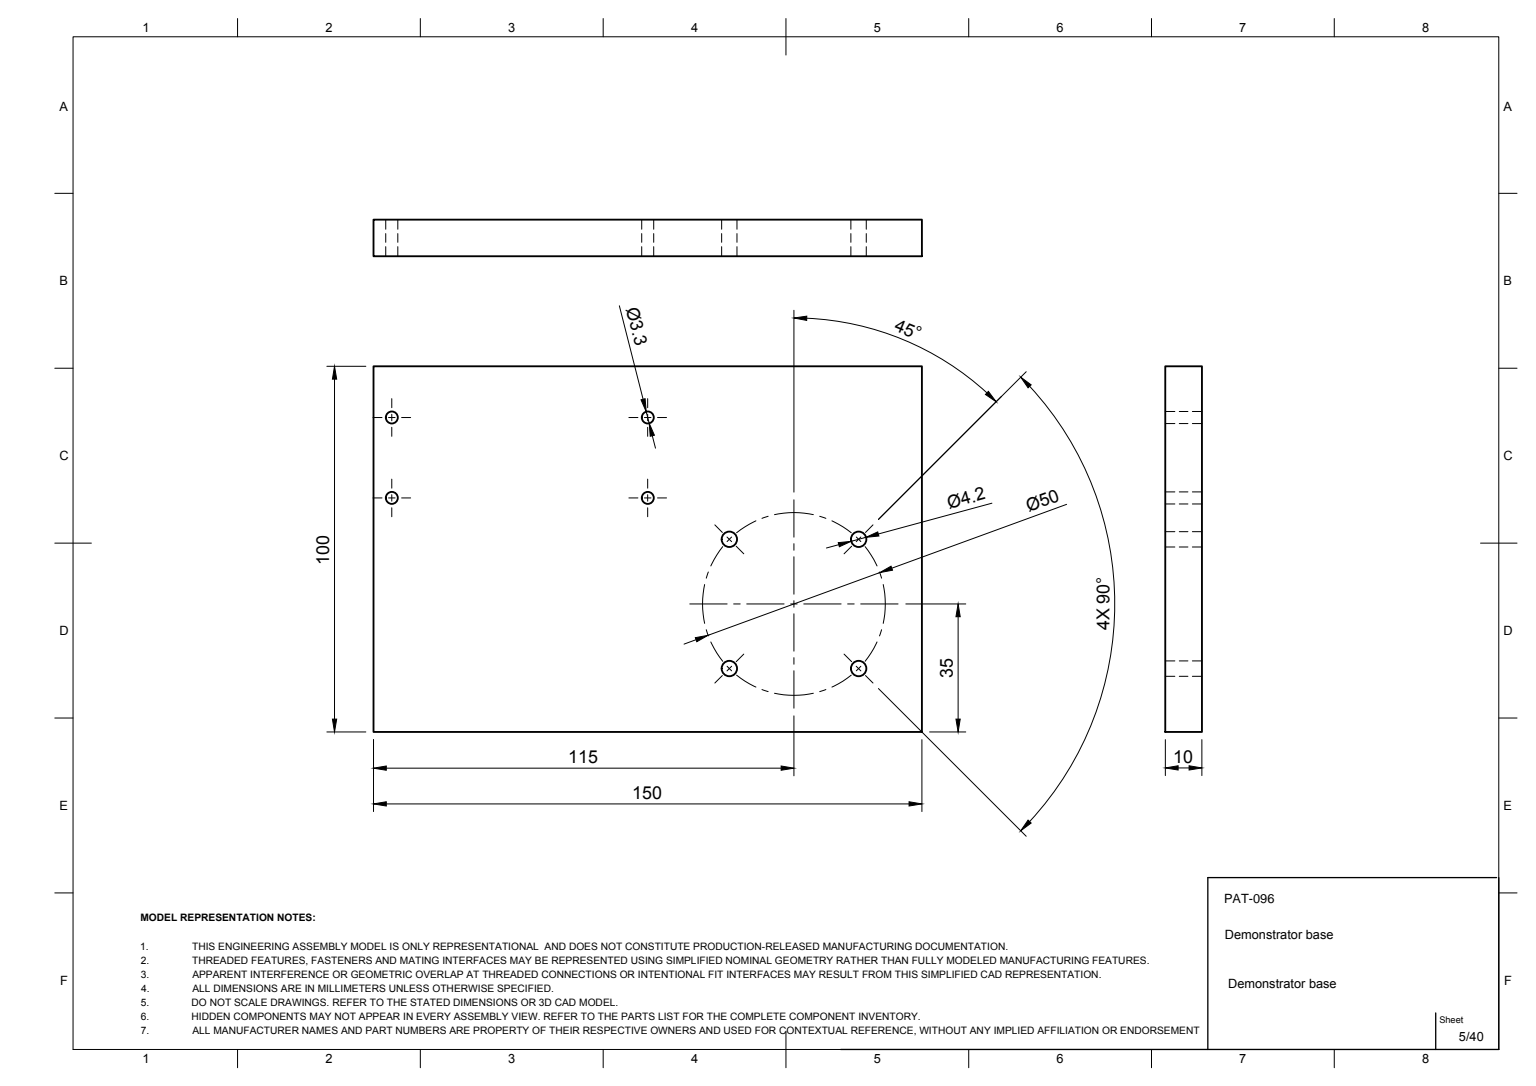
ISO-10303-21;
HEADER;
/* Generated by software containing ST-Developer
 * from STEP Tools, Inc. (www.steptools.com) 
 */

FILE_DESCRIPTION(
/* description */ ('PAT-096'),
/* implementation_level */ '2;1');

FILE_NAME(
/* name */ 'Demonstrator base.step',
/* time_stamp */ '2026-10-29T17:03:14-07:00',
/* author */ (''),
/* organization */ (''),
/* preprocessor_version */ 'ST-DEVELOPER v20.2',
/* originating_system */ 'Autodesk Translation Framework v15.17.0.0',
/* authorisation */ '');

FILE_SCHEMA (('AUTOMOTIVE_DESIGN { 1 0 10303 214 3 1 1 }'));
ENDSEC;

DATA;
#10=MECHANICAL_DESIGN_GEOMETRIC_PRESENTATION_REPRESENTATION('',(#398),#10650);
#336=SHAPE_REPRESENTATION_RELATIONSHIP('SRR','None',#10796,#367);
#367=ADVANCED_BREP_SHAPE_REPRESENTATION('',(#437),#10614);
#398=STYLED_ITEM('',(#11043),#437);
#437=MANIFOLD_SOLID_BREP('Body1',#5531);
#473=FACE_BOUND('',#1139,.T.);
#474=FACE_BOUND('',#1140,.T.);
#475=FACE_BOUND('',#1141,.T.);
#476=FACE_BOUND('',#1142,.T.);
#477=FACE_BOUND('',#1143,.T.);
#478=FACE_BOUND('',#1144,.T.);
#479=FACE_BOUND('',#1145,.T.);
#480=FACE_BOUND('',#1146,.T.);
#481=FACE_BOUND('',#1148,.T.);
#482=FACE_BOUND('',#1149,.T.);
#483=FACE_BOUND('',#1150,.T.);
#484=FACE_BOUND('',#1151,.T.);
#485=FACE_BOUND('',#1152,.T.);
#486=FACE_BOUND('',#1153,.T.);
#487=FACE_BOUND('',#1154,.T.);
#488=FACE_BOUND('',#1155,.T.);
#612=PLANE('',#5942);
#613=PLANE('',#5943);
#614=PLANE('',#5944);
#615=PLANE('',#5945);
#616=PLANE('',#5946);
#617=PLANE('',#5947);
#790=FACE_OUTER_BOUND('',#1126,.T.);
#791=FACE_OUTER_BOUND('',#1127,.T.);
#792=FACE_OUTER_BOUND('',#1128,.T.);
#793=FACE_OUTER_BOUND('',#1129,.T.);
#794=FACE_OUTER_BOUND('',#1130,.T.);
#795=FACE_OUTER_BOUND('',#1131,.T.);
#796=FACE_OUTER_BOUND('',#1132,.T.);
#797=FACE_OUTER_BOUND('',#1133,.T.);
#798=FACE_OUTER_BOUND('',#1134,.T.);
#799=FACE_OUTER_BOUND('',#1135,.T.);
#800=FACE_OUTER_BOUND('',#1136,.T.);
#801=FACE_OUTER_BOUND('',#1137,.T.);
#802=FACE_OUTER_BOUND('',#1138,.T.);
#803=FACE_OUTER_BOUND('',#1147,.T.);
#1126=EDGE_LOOP('',(#3715,#3716,#3717,#3718));
#1127=EDGE_LOOP('',(#3719,#3720,#3721,#3722));
#1128=EDGE_LOOP('',(#3723,#3724,#3725,#3726));
#1129=EDGE_LOOP('',(#3727,#3728,#3729,#3730));
#1130=EDGE_LOOP('',(#3731,#3732,#3733,#3734));
#1131=EDGE_LOOP('',(#3735,#3736,#3737,#3738));
#1132=EDGE_LOOP('',(#3739,#3740,#3741,#3742));
#1133=EDGE_LOOP('',(#3743,#3744,#3745,#3746));
#1134=EDGE_LOOP('',(#3747,#3748,#3749,#3750));
#1135=EDGE_LOOP('',(#3751,#3752,#3753,#3754));
#1136=EDGE_LOOP('',(#3755,#3756,#3757,#3758));
#1137=EDGE_LOOP('',(#3759,#3760,#3761,#3762));
#1138=EDGE_LOOP('',(#3763,#3764,#3765,#3766));
#1139=EDGE_LOOP('',(#3767));
#1140=EDGE_LOOP('',(#3768));
#1141=EDGE_LOOP('',(#3769));
#1142=EDGE_LOOP('',(#3770));
#1143=EDGE_LOOP('',(#3771));
#1144=EDGE_LOOP('',(#3772));
#1145=EDGE_LOOP('',(#3773));
#1146=EDGE_LOOP('',(#3774));
#1147=EDGE_LOOP('',(#3775,#3776,#3777,#3778));
#1148=EDGE_LOOP('',(#3779));
#1149=EDGE_LOOP('',(#3780));
#1150=EDGE_LOOP('',(#3781));
#1151=EDGE_LOOP('',(#3782));
#1152=EDGE_LOOP('',(#3783));
#1153=EDGE_LOOP('',(#3784));
#1154=EDGE_LOOP('',(#3785));
#1155=EDGE_LOOP('',(#3786));
#1601=LINE('',#8519,#1930);
#1602=LINE('',#8525,#1931);
#1603=LINE('',#8531,#1932);
#1604=LINE('',#8537,#1933);
#1605=LINE('',#8543,#1934);
#1606=LINE('',#8549,#1935);
#1607=LINE('',#8555,#1936);
#1608=LINE('',#8561,#1937);
#1609=LINE('',#8566,#1938);
#1610=LINE('',#8568,#1939);
#1611=LINE('',#8570,#1940);
#1612=LINE('',#8571,#1941);
#1613=LINE('',#8574,#1942);
#1614=LINE('',#8576,#1943);
#1615=LINE('',#8577,#1944);
#1616=LINE('',#8580,#1945);
#1617=LINE('',#8582,#1946);
#1618=LINE('',#8583,#1947);
#1619=LINE('',#8585,#1948);
#1620=LINE('',#8586,#1949);
#1930=VECTOR('',#6681,0.164999999999999);
#1931=VECTOR('',#6688,0.164999999999999);
#1932=VECTOR('',#6695,0.165);
#1933=VECTOR('',#6702,0.165);
#1934=VECTOR('',#6709,0.21);
#1935=VECTOR('',#6716,0.21);
#1936=VECTOR('',#6723,0.21);
#1937=VECTOR('',#6730,0.21);
#1938=VECTOR('',#6735,1.);
#1939=VECTOR('',#6736,1.);
#1940=VECTOR('',#6737,1.);
#1941=VECTOR('',#6738,1.);
#1942=VECTOR('',#6741,1.);
#1943=VECTOR('',#6742,1.);
#1944=VECTOR('',#6743,1.);
#1945=VECTOR('',#6746,1.);
#1946=VECTOR('',#6747,1.);
#1947=VECTOR('',#6748,1.);
#1948=VECTOR('',#6751,1.);
#1949=VECTOR('',#6752,1.);
#2259=CIRCLE('',#5919,0.164999999999999);
#2260=CIRCLE('',#5920,0.164999999999999);
#2261=CIRCLE('',#5922,0.164999999999999);
#2262=CIRCLE('',#5923,0.164999999999999);
#2263=CIRCLE('',#5925,0.165);
#2264=CIRCLE('',#5926,0.165);
#2265=CIRCLE('',#5928,0.165);
#2266=CIRCLE('',#5929,0.165);
#2267=CIRCLE('',#5931,0.21);
#2268=CIRCLE('',#5932,0.21);
#2269=CIRCLE('',#5934,0.21);
#2270=CIRCLE('',#5935,0.21);
#2271=CIRCLE('',#5937,0.21);
#2272=CIRCLE('',#5938,0.21);
#2273=CIRCLE('',#5940,0.21);
#2274=CIRCLE('',#5941,0.21);
#2578=VERTEX_POINT('',#8516);
#2579=VERTEX_POINT('',#8518);
#2580=VERTEX_POINT('',#8522);
#2581=VERTEX_POINT('',#8524);
#2582=VERTEX_POINT('',#8528);
#2583=VERTEX_POINT('',#8530);
#2584=VERTEX_POINT('',#8534);
#2585=VERTEX_POINT('',#8536);
#2586=VERTEX_POINT('',#8540);
#2587=VERTEX_POINT('',#8542);
#2588=VERTEX_POINT('',#8546);
#2589=VERTEX_POINT('',#8548);
#2590=VERTEX_POINT('',#8552);
#2591=VERTEX_POINT('',#8554);
#2592=VERTEX_POINT('',#8558);
#2593=VERTEX_POINT('',#8560);
#2594=VERTEX_POINT('',#8564);
#2595=VERTEX_POINT('',#8565);
#2596=VERTEX_POINT('',#8567);
#2597=VERTEX_POINT('',#8569);
#2598=VERTEX_POINT('',#8573);
#2599=VERTEX_POINT('',#8575);
#2600=VERTEX_POINT('',#8579);
#2601=VERTEX_POINT('',#8581);
#3036=EDGE_CURVE('',#2578,#2578,#2259,.T.);
#3037=EDGE_CURVE('',#2578,#2579,#1601,.T.);
#3038=EDGE_CURVE('',#2579,#2579,#2260,.T.);
#3039=EDGE_CURVE('',#2580,#2580,#2261,.T.);
#3040=EDGE_CURVE('',#2580,#2581,#1602,.T.);
#3041=EDGE_CURVE('',#2581,#2581,#2262,.T.);
#3042=EDGE_CURVE('',#2582,#2582,#2263,.T.);
#3043=EDGE_CURVE('',#2582,#2583,#1603,.T.);
#3044=EDGE_CURVE('',#2583,#2583,#2264,.T.);
#3045=EDGE_CURVE('',#2584,#2584,#2265,.T.);
#3046=EDGE_CURVE('',#2584,#2585,#1604,.T.);
#3047=EDGE_CURVE('',#2585,#2585,#2266,.T.);
#3048=EDGE_CURVE('',#2586,#2586,#2267,.T.);
#3049=EDGE_CURVE('',#2586,#2587,#1605,.T.);
#3050=EDGE_CURVE('',#2587,#2587,#2268,.T.);
#3051=EDGE_CURVE('',#2588,#2588,#2269,.T.);
#3052=EDGE_CURVE('',#2588,#2589,#1606,.T.);
#3053=EDGE_CURVE('',#2589,#2589,#2270,.T.);
#3054=EDGE_CURVE('',#2590,#2590,#2271,.T.);
#3055=EDGE_CURVE('',#2590,#2591,#1607,.T.);
#3056=EDGE_CURVE('',#2591,#2591,#2272,.T.);
#3057=EDGE_CURVE('',#2592,#2592,#2273,.T.);
#3058=EDGE_CURVE('',#2592,#2593,#1608,.T.);
#3059=EDGE_CURVE('',#2593,#2593,#2274,.T.);
#3060=EDGE_CURVE('',#2594,#2595,#1609,.T.);
#3061=EDGE_CURVE('',#2595,#2596,#1610,.T.);
#3062=EDGE_CURVE('',#2597,#2596,#1611,.T.);
#3063=EDGE_CURVE('',#2594,#2597,#1612,.T.);
#3064=EDGE_CURVE('',#2598,#2594,#1613,.T.);
#3065=EDGE_CURVE('',#2599,#2597,#1614,.T.);
#3066=EDGE_CURVE('',#2598,#2599,#1615,.T.);
#3067=EDGE_CURVE('',#2600,#2598,#1616,.T.);
#3068=EDGE_CURVE('',#2601,#2599,#1617,.T.);
#3069=EDGE_CURVE('',#2600,#2601,#1618,.T.);
#3070=EDGE_CURVE('',#2595,#2600,#1619,.T.);
#3071=EDGE_CURVE('',#2596,#2601,#1620,.T.);
#3715=ORIENTED_EDGE('',*,*,#3036,.F.);
#3716=ORIENTED_EDGE('',*,*,#3037,.T.);
#3717=ORIENTED_EDGE('',*,*,#3038,.F.);
#3718=ORIENTED_EDGE('',*,*,#3037,.F.);
#3719=ORIENTED_EDGE('',*,*,#3039,.F.);
#3720=ORIENTED_EDGE('',*,*,#3040,.T.);
#3721=ORIENTED_EDGE('',*,*,#3041,.F.);
#3722=ORIENTED_EDGE('',*,*,#3040,.F.);
#3723=ORIENTED_EDGE('',*,*,#3042,.F.);
#3724=ORIENTED_EDGE('',*,*,#3043,.T.);
#3725=ORIENTED_EDGE('',*,*,#3044,.F.);
#3726=ORIENTED_EDGE('',*,*,#3043,.F.);
#3727=ORIENTED_EDGE('',*,*,#3045,.F.);
#3728=ORIENTED_EDGE('',*,*,#3046,.T.);
#3729=ORIENTED_EDGE('',*,*,#3047,.F.);
#3730=ORIENTED_EDGE('',*,*,#3046,.F.);
#3731=ORIENTED_EDGE('',*,*,#3048,.F.);
#3732=ORIENTED_EDGE('',*,*,#3049,.T.);
#3733=ORIENTED_EDGE('',*,*,#3050,.F.);
#3734=ORIENTED_EDGE('',*,*,#3049,.F.);
#3735=ORIENTED_EDGE('',*,*,#3051,.F.);
#3736=ORIENTED_EDGE('',*,*,#3052,.T.);
#3737=ORIENTED_EDGE('',*,*,#3053,.F.);
#3738=ORIENTED_EDGE('',*,*,#3052,.F.);
#3739=ORIENTED_EDGE('',*,*,#3054,.F.);
#3740=ORIENTED_EDGE('',*,*,#3055,.T.);
#3741=ORIENTED_EDGE('',*,*,#3056,.F.);
#3742=ORIENTED_EDGE('',*,*,#3055,.F.);
#3743=ORIENTED_EDGE('',*,*,#3057,.F.);
#3744=ORIENTED_EDGE('',*,*,#3058,.T.);
#3745=ORIENTED_EDGE('',*,*,#3059,.F.);
#3746=ORIENTED_EDGE('',*,*,#3058,.F.);
#3747=ORIENTED_EDGE('',*,*,#3060,.T.);
#3748=ORIENTED_EDGE('',*,*,#3061,.T.);
#3749=ORIENTED_EDGE('',*,*,#3062,.F.);
#3750=ORIENTED_EDGE('',*,*,#3063,.F.);
#3751=ORIENTED_EDGE('',*,*,#3064,.T.);
#3752=ORIENTED_EDGE('',*,*,#3063,.T.);
#3753=ORIENTED_EDGE('',*,*,#3065,.F.);
#3754=ORIENTED_EDGE('',*,*,#3066,.F.);
#3755=ORIENTED_EDGE('',*,*,#3067,.T.);
#3756=ORIENTED_EDGE('',*,*,#3066,.T.);
#3757=ORIENTED_EDGE('',*,*,#3068,.F.);
#3758=ORIENTED_EDGE('',*,*,#3069,.F.);
#3759=ORIENTED_EDGE('',*,*,#3070,.T.);
#3760=ORIENTED_EDGE('',*,*,#3069,.T.);
#3761=ORIENTED_EDGE('',*,*,#3071,.F.);
#3762=ORIENTED_EDGE('',*,*,#3061,.F.);
#3763=ORIENTED_EDGE('',*,*,#3071,.T.);
#3764=ORIENTED_EDGE('',*,*,#3068,.T.);
#3765=ORIENTED_EDGE('',*,*,#3065,.T.);
#3766=ORIENTED_EDGE('',*,*,#3062,.T.);
#3767=ORIENTED_EDGE('',*,*,#3059,.T.);
#3768=ORIENTED_EDGE('',*,*,#3056,.T.);
#3769=ORIENTED_EDGE('',*,*,#3053,.T.);
#3770=ORIENTED_EDGE('',*,*,#3050,.T.);
#3771=ORIENTED_EDGE('',*,*,#3047,.T.);
#3772=ORIENTED_EDGE('',*,*,#3044,.T.);
#3773=ORIENTED_EDGE('',*,*,#3041,.T.);
#3774=ORIENTED_EDGE('',*,*,#3038,.T.);
#3775=ORIENTED_EDGE('',*,*,#3070,.F.);
#3776=ORIENTED_EDGE('',*,*,#3060,.F.);
#3777=ORIENTED_EDGE('',*,*,#3064,.F.);
#3778=ORIENTED_EDGE('',*,*,#3067,.F.);
#3779=ORIENTED_EDGE('',*,*,#3057,.T.);
#3780=ORIENTED_EDGE('',*,*,#3054,.T.);
#3781=ORIENTED_EDGE('',*,*,#3051,.T.);
#3782=ORIENTED_EDGE('',*,*,#3048,.T.);
#3783=ORIENTED_EDGE('',*,*,#3045,.T.);
#3784=ORIENTED_EDGE('',*,*,#3042,.T.);
#3785=ORIENTED_EDGE('',*,*,#3039,.T.);
#3786=ORIENTED_EDGE('',*,*,#3036,.T.);
#5073=CYLINDRICAL_SURFACE('',#5918,0.164999999999999);
#5074=CYLINDRICAL_SURFACE('',#5921,0.164999999999999);
#5075=CYLINDRICAL_SURFACE('',#5924,0.165);
#5076=CYLINDRICAL_SURFACE('',#5927,0.165);
#5077=CYLINDRICAL_SURFACE('',#5930,0.21);
#5078=CYLINDRICAL_SURFACE('',#5933,0.21);
#5079=CYLINDRICAL_SURFACE('',#5936,0.21);
#5080=CYLINDRICAL_SURFACE('',#5939,0.21);
#5195=ADVANCED_FACE('',(#790),#5073,.F.);
#5196=ADVANCED_FACE('',(#791),#5074,.F.);
#5197=ADVANCED_FACE('',(#792),#5075,.F.);
#5198=ADVANCED_FACE('',(#793),#5076,.F.);
#5199=ADVANCED_FACE('',(#794),#5077,.F.);
#5200=ADVANCED_FACE('',(#795),#5078,.F.);
#5201=ADVANCED_FACE('',(#796),#5079,.F.);
#5202=ADVANCED_FACE('',(#797),#5080,.F.);
#5203=ADVANCED_FACE('',(#798),#612,.T.);
#5204=ADVANCED_FACE('',(#799),#613,.T.);
#5205=ADVANCED_FACE('',(#800),#614,.T.);
#5206=ADVANCED_FACE('',(#801),#615,.T.);
#5207=ADVANCED_FACE('',(#802,#473,#474,#475,#476,#477,#478,#479,#480),#616,
 .T.);
#5208=ADVANCED_FACE('',(#803,#481,#482,#483,#484,#485,#486,#487,#488),#617,
 .F.);
#5531=CLOSED_SHELL('',(#5195,#5196,#5197,#5198,#5199,#5200,#5201,#5202,
#5203,#5204,#5205,#5206,#5207,#5208));
#5917=AXIS2_PLACEMENT_3D('',#8514,#6675,#6676);
#5918=AXIS2_PLACEMENT_3D('',#8515,#6677,#6678);
#5919=AXIS2_PLACEMENT_3D('',#8517,#6679,#6680);
#5920=AXIS2_PLACEMENT_3D('',#8520,#6682,#6683);
#5921=AXIS2_PLACEMENT_3D('',#8521,#6684,#6685);
#5922=AXIS2_PLACEMENT_3D('',#8523,#6686,#6687);
#5923=AXIS2_PLACEMENT_3D('',#8526,#6689,#6690);
#5924=AXIS2_PLACEMENT_3D('',#8527,#6691,#6692);
#5925=AXIS2_PLACEMENT_3D('',#8529,#6693,#6694);
#5926=AXIS2_PLACEMENT_3D('',#8532,#6696,#6697);
#5927=AXIS2_PLACEMENT_3D('',#8533,#6698,#6699);
#5928=AXIS2_PLACEMENT_3D('',#8535,#6700,#6701);
#5929=AXIS2_PLACEMENT_3D('',#8538,#6703,#6704);
#5930=AXIS2_PLACEMENT_3D('',#8539,#6705,#6706);
#5931=AXIS2_PLACEMENT_3D('',#8541,#6707,#6708);
#5932=AXIS2_PLACEMENT_3D('',#8544,#6710,#6711);
#5933=AXIS2_PLACEMENT_3D('',#8545,#6712,#6713);
#5934=AXIS2_PLACEMENT_3D('',#8547,#6714,#6715);
#5935=AXIS2_PLACEMENT_3D('',#8550,#6717,#6718);
#5936=AXIS2_PLACEMENT_3D('',#8551,#6719,#6720);
#5937=AXIS2_PLACEMENT_3D('',#8553,#6721,#6722);
#5938=AXIS2_PLACEMENT_3D('',#8556,#6724,#6725);
#5939=AXIS2_PLACEMENT_3D('',#8557,#6726,#6727);
#5940=AXIS2_PLACEMENT_3D('',#8559,#6728,#6729);
#5941=AXIS2_PLACEMENT_3D('',#8562,#6731,#6732);
#5942=AXIS2_PLACEMENT_3D('',#8563,#6733,#6734);
#5943=AXIS2_PLACEMENT_3D('',#8572,#6739,#6740);
#5944=AXIS2_PLACEMENT_3D('',#8578,#6744,#6745);
#5945=AXIS2_PLACEMENT_3D('',#8584,#6749,#6750);
#5946=AXIS2_PLACEMENT_3D('',#8587,#6753,#6754);
#5947=AXIS2_PLACEMENT_3D('',#8588,#6755,#6756);
#6675=DIRECTION('axis',(0.,0.,1.));
#6676=DIRECTION('refdir',(1.,0.,0.));
#6677=DIRECTION('center_axis',(0.,0.,1.));
#6678=DIRECTION('ref_axis',(1.,0.,0.));
#6679=DIRECTION('center_axis',(0.,0.,1.));
#6680=DIRECTION('ref_axis',(1.,0.,0.));
#6681=DIRECTION('',(0.,0.,1.));
#6682=DIRECTION('center_axis',(0.,0.,-1.));
#6683=DIRECTION('ref_axis',(1.,0.,0.));
#6684=DIRECTION('center_axis',(0.,0.,1.));
#6685=DIRECTION('ref_axis',(1.,0.,0.));
#6686=DIRECTION('center_axis',(0.,0.,1.));
#6687=DIRECTION('ref_axis',(1.,0.,0.));
#6688=DIRECTION('',(0.,0.,1.));
#6689=DIRECTION('center_axis',(0.,0.,-1.));
#6690=DIRECTION('ref_axis',(1.,0.,0.));
#6691=DIRECTION('center_axis',(0.,0.,1.));
#6692=DIRECTION('ref_axis',(1.,0.,0.));
#6693=DIRECTION('center_axis',(0.,0.,1.));
#6694=DIRECTION('ref_axis',(1.,0.,0.));
#6695=DIRECTION('',(0.,0.,1.));
#6696=DIRECTION('center_axis',(0.,0.,-1.));
#6697=DIRECTION('ref_axis',(1.,0.,0.));
#6698=DIRECTION('center_axis',(0.,0.,1.));
#6699=DIRECTION('ref_axis',(1.,0.,0.));
#6700=DIRECTION('center_axis',(0.,0.,1.));
#6701=DIRECTION('ref_axis',(1.,0.,0.));
#6702=DIRECTION('',(0.,0.,1.));
#6703=DIRECTION('center_axis',(0.,0.,-1.));
#6704=DIRECTION('ref_axis',(1.,0.,0.));
#6705=DIRECTION('center_axis',(0.,0.,1.));
#6706=DIRECTION('ref_axis',(1.,0.,0.));
#6707=DIRECTION('center_axis',(0.,0.,1.));
#6708=DIRECTION('ref_axis',(1.,0.,0.));
#6709=DIRECTION('',(0.,0.,1.));
#6710=DIRECTION('center_axis',(0.,0.,-1.));
#6711=DIRECTION('ref_axis',(1.,0.,0.));
#6712=DIRECTION('center_axis',(0.,0.,1.));
#6713=DIRECTION('ref_axis',(1.,0.,0.));
#6714=DIRECTION('center_axis',(0.,0.,1.));
#6715=DIRECTION('ref_axis',(1.,0.,0.));
#6716=DIRECTION('',(0.,0.,1.));
#6717=DIRECTION('center_axis',(0.,0.,-1.));
#6718=DIRECTION('ref_axis',(1.,0.,0.));
#6719=DIRECTION('center_axis',(0.,0.,1.));
#6720=DIRECTION('ref_axis',(1.,0.,0.));
#6721=DIRECTION('center_axis',(0.,0.,1.));
#6722=DIRECTION('ref_axis',(1.,0.,0.));
#6723=DIRECTION('',(0.,0.,1.));
#6724=DIRECTION('center_axis',(0.,0.,-1.));
#6725=DIRECTION('ref_axis',(1.,0.,0.));
#6726=DIRECTION('center_axis',(0.,0.,1.));
#6727=DIRECTION('ref_axis',(1.,0.,0.));
#6728=DIRECTION('center_axis',(0.,0.,1.));
#6729=DIRECTION('ref_axis',(1.,0.,0.));
#6730=DIRECTION('',(0.,0.,1.));
#6731=DIRECTION('center_axis',(0.,0.,-1.));
#6732=DIRECTION('ref_axis',(1.,0.,0.));
#6733=DIRECTION('center_axis',(0.,1.,0.));
#6734=DIRECTION('ref_axis',(-1.,0.,0.));
#6735=DIRECTION('',(-1.,0.,0.));
#6736=DIRECTION('',(0.,0.,1.));
#6737=DIRECTION('',(-1.,0.,0.));
#6738=DIRECTION('',(0.,0.,1.));
#6739=DIRECTION('center_axis',(1.,0.,0.));
#6740=DIRECTION('ref_axis',(0.,1.,0.));
#6741=DIRECTION('',(0.,1.,0.));
#6742=DIRECTION('',(0.,1.,0.));
#6743=DIRECTION('',(0.,0.,1.));
#6744=DIRECTION('center_axis',(0.,-1.,0.));
#6745=DIRECTION('ref_axis',(1.,0.,0.));
#6746=DIRECTION('',(1.,0.,0.));
#6747=DIRECTION('',(1.,0.,0.));
#6748=DIRECTION('',(0.,0.,1.));
#6749=DIRECTION('center_axis',(-1.,0.,0.));
#6750=DIRECTION('ref_axis',(0.,-1.,0.));
#6751=DIRECTION('',(0.,-1.,0.));
#6752=DIRECTION('',(0.,-1.,0.));
#6753=DIRECTION('center_axis',(0.,0.,1.));
#6754=DIRECTION('ref_axis',(1.,0.,0.));
#6755=DIRECTION('center_axis',(0.,0.,1.));
#6756=DIRECTION('ref_axis',(1.,0.,0.));
#8514=CARTESIAN_POINT('',(0.,0.,0.));
#8515=CARTESIAN_POINT('Origin',(11.,2.9,-0.1));
#8516=CARTESIAN_POINT('',(10.835,2.9,0.));
#8517=CARTESIAN_POINT('Origin',(11.,2.9,0.));
#8518=CARTESIAN_POINT('',(10.835,2.9,1.));
#8519=CARTESIAN_POINT('',(10.835,2.9,-0.1));
#8520=CARTESIAN_POINT('Origin',(11.,2.9,1.));
#8521=CARTESIAN_POINT('Origin',(11.,5.1,-0.1));
#8522=CARTESIAN_POINT('',(10.835,5.1,0.));
#8523=CARTESIAN_POINT('Origin',(11.,5.1,0.));
#8524=CARTESIAN_POINT('',(10.835,5.1,1.));
#8525=CARTESIAN_POINT('',(10.835,5.1,-0.1));
#8526=CARTESIAN_POINT('Origin',(11.,5.1,1.));
#8527=CARTESIAN_POINT('Origin',(4.,2.9,-0.1));
#8528=CARTESIAN_POINT('',(3.835,2.9,0.));
#8529=CARTESIAN_POINT('Origin',(4.,2.9,0.));
#8530=CARTESIAN_POINT('',(3.835,2.9,1.));
#8531=CARTESIAN_POINT('',(3.835,2.9,-0.1));
#8532=CARTESIAN_POINT('Origin',(4.,2.9,1.));
#8533=CARTESIAN_POINT('Origin',(4.,5.1,-0.1));
#8534=CARTESIAN_POINT('',(3.835,5.1,0.));
#8535=CARTESIAN_POINT('Origin',(4.,5.1,0.));
#8536=CARTESIAN_POINT('',(3.835,5.1,1.));
#8537=CARTESIAN_POINT('',(3.835,5.1,-0.1));
#8538=CARTESIAN_POINT('Origin',(4.,5.1,1.));
#8539=CARTESIAN_POINT('Origin',(-1.76776695296637,-1.76776695296637,-0.1));
#8540=CARTESIAN_POINT('',(-1.97776695296637,-1.76776695296637,0.));
#8541=CARTESIAN_POINT('Origin',(-1.76776695296637,-1.76776695296637,0.));
#8542=CARTESIAN_POINT('',(-1.97776695296637,-1.76776695296637,1.));
#8543=CARTESIAN_POINT('',(-1.97776695296637,-1.76776695296637,-0.1));
#8544=CARTESIAN_POINT('Origin',(-1.76776695296637,-1.76776695296637,1.));
#8545=CARTESIAN_POINT('Origin',(-1.76776695296637,1.76776695296637,-0.1));
#8546=CARTESIAN_POINT('',(-1.97776695296637,1.76776695296637,0.));
#8547=CARTESIAN_POINT('Origin',(-1.76776695296637,1.76776695296637,0.));
#8548=CARTESIAN_POINT('',(-1.97776695296637,1.76776695296637,1.));
#8549=CARTESIAN_POINT('',(-1.97776695296637,1.76776695296637,-0.1));
#8550=CARTESIAN_POINT('Origin',(-1.76776695296637,1.76776695296637,1.));
#8551=CARTESIAN_POINT('Origin',(1.76776695296637,1.76776695296637,-0.1));
#8552=CARTESIAN_POINT('',(1.55776695296637,1.76776695296637,0.));
#8553=CARTESIAN_POINT('Origin',(1.76776695296637,1.76776695296637,0.));
#8554=CARTESIAN_POINT('',(1.55776695296637,1.76776695296637,1.));
#8555=CARTESIAN_POINT('',(1.55776695296637,1.76776695296637,-0.1));
#8556=CARTESIAN_POINT('Origin',(1.76776695296637,1.76776695296637,1.));
#8557=CARTESIAN_POINT('Origin',(1.76776695296637,-1.76776695296637,-0.1));
#8558=CARTESIAN_POINT('',(1.55776695296637,-1.76776695296637,0.));
#8559=CARTESIAN_POINT('Origin',(1.76776695296637,-1.76776695296637,0.));
#8560=CARTESIAN_POINT('',(1.55776695296637,-1.76776695296637,1.));
#8561=CARTESIAN_POINT('',(1.55776695296637,-1.76776695296637,-0.1));
#8562=CARTESIAN_POINT('Origin',(1.76776695296637,-1.76776695296637,1.));
#8563=CARTESIAN_POINT('Origin',(11.5,6.5,0.));
#8564=CARTESIAN_POINT('',(11.5,6.5,0.));
#8565=CARTESIAN_POINT('',(-3.5,6.5,0.));
#8566=CARTESIAN_POINT('',(11.5,6.5,0.));
#8567=CARTESIAN_POINT('',(-3.5,6.5,1.));
#8568=CARTESIAN_POINT('',(-3.5,6.5,0.));
#8569=CARTESIAN_POINT('',(11.5,6.5,1.));
#8570=CARTESIAN_POINT('',(11.5,6.5,1.));
#8571=CARTESIAN_POINT('',(11.5,6.5,0.));
#8572=CARTESIAN_POINT('Origin',(11.5,-3.5,0.));
#8573=CARTESIAN_POINT('',(11.5,-3.5,0.));
#8574=CARTESIAN_POINT('',(11.5,-3.5,0.));
#8575=CARTESIAN_POINT('',(11.5,-3.5,1.));
#8576=CARTESIAN_POINT('',(11.5,-3.5,1.));
#8577=CARTESIAN_POINT('',(11.5,-3.5,0.));
#8578=CARTESIAN_POINT('Origin',(-3.5,-3.5,0.));
#8579=CARTESIAN_POINT('',(-3.5,-3.5,0.));
#8580=CARTESIAN_POINT('',(-3.5,-3.5,0.));
#8581=CARTESIAN_POINT('',(-3.5,-3.5,1.));
#8582=CARTESIAN_POINT('',(-3.5,-3.5,1.));
#8583=CARTESIAN_POINT('',(-3.5,-3.5,0.));
#8584=CARTESIAN_POINT('Origin',(-3.5,6.5,0.));
#8585=CARTESIAN_POINT('',(-3.5,6.5,0.));
#8586=CARTESIAN_POINT('',(-3.5,6.5,1.));
#8587=CARTESIAN_POINT('Origin',(4.,1.5,1.));
#8588=CARTESIAN_POINT('Origin',(4.,1.5,0.));
#10575=UNCERTAINTY_MEASURE_WITH_UNIT(LENGTH_MEASURE(0.001),#10651,
'DISTANCE_ACCURACY_VALUE',
'Maximum model space distance between geometric entities at asserted c
onnectivities');
#10611=UNCERTAINTY_MEASURE_WITH_UNIT(LENGTH_MEASURE(0.001),#10651,
'DISTANCE_ACCURACY_VALUE',
'Maximum model space distance between geometric entities at asserted c
onnectivities');
#10614=(
GEOMETRIC_REPRESENTATION_CONTEXT(3)
GLOBAL_UNCERTAINTY_ASSIGNED_CONTEXT((#10575))
GLOBAL_UNIT_ASSIGNED_CONTEXT((#10651,#10653,#10654))
REPRESENTATION_CONTEXT('','3D')
);
#10650=(
GEOMETRIC_REPRESENTATION_CONTEXT(3)
GLOBAL_UNCERTAINTY_ASSIGNED_CONTEXT((#10611))
GLOBAL_UNIT_ASSIGNED_CONTEXT((#10651,#10653,#10654))
REPRESENTATION_CONTEXT('','3D')
);
#10651=(
LENGTH_UNIT()
NAMED_UNIT(*)
SI_UNIT(.CENTI.,.METRE.)
);
#10653=(
NAMED_UNIT(*)
PLANE_ANGLE_UNIT()
SI_UNIT($,.RADIAN.)
);
#10654=(
NAMED_UNIT(*)
SI_UNIT($,.STERADIAN.)
SOLID_ANGLE_UNIT()
);
#10657=SHAPE_DEFINITION_REPRESENTATION(#10695,#10796);
#10695=PRODUCT_DEFINITION_SHAPE('',$,#10835);
#10796=SHAPE_REPRESENTATION('',(#5917),#10614);
#10832=PRODUCT_DEFINITION_CONTEXT('part definition',#10948,'design');
#10835=PRODUCT_DEFINITION('Demonstrator base','Demonstrator base',#10873,
#10832);
#10873=PRODUCT_DEFINITION_FORMATION('',$,#10952);
#10948=APPLICATION_CONTEXT(
'Core Data for Automotive Mechanical Design Process');
#10949=PRODUCT_CONTEXT('part definition',#10948,'mechanical');
#10952=PRODUCT('Demonstrator base','Demonstrator base',
'Demonstrator base',(#10949));
#11037=COLOUR_RGB('Dark Blue',0.08,0.2,0.34);
#11038=FILL_AREA_STYLE_COLOUR('',#11037);
#11039=FILL_AREA_STYLE('',(#11038));
#11040=SURFACE_STYLE_FILL_AREA(#11039);
#11041=SURFACE_SIDE_STYLE('',(#11040));
#11042=SURFACE_STYLE_USAGE(.BOTH.,#11041);
#11043=PRESENTATION_STYLE_ASSIGNMENT((#11042));
ENDSEC;
END-ISO-10303-21;
